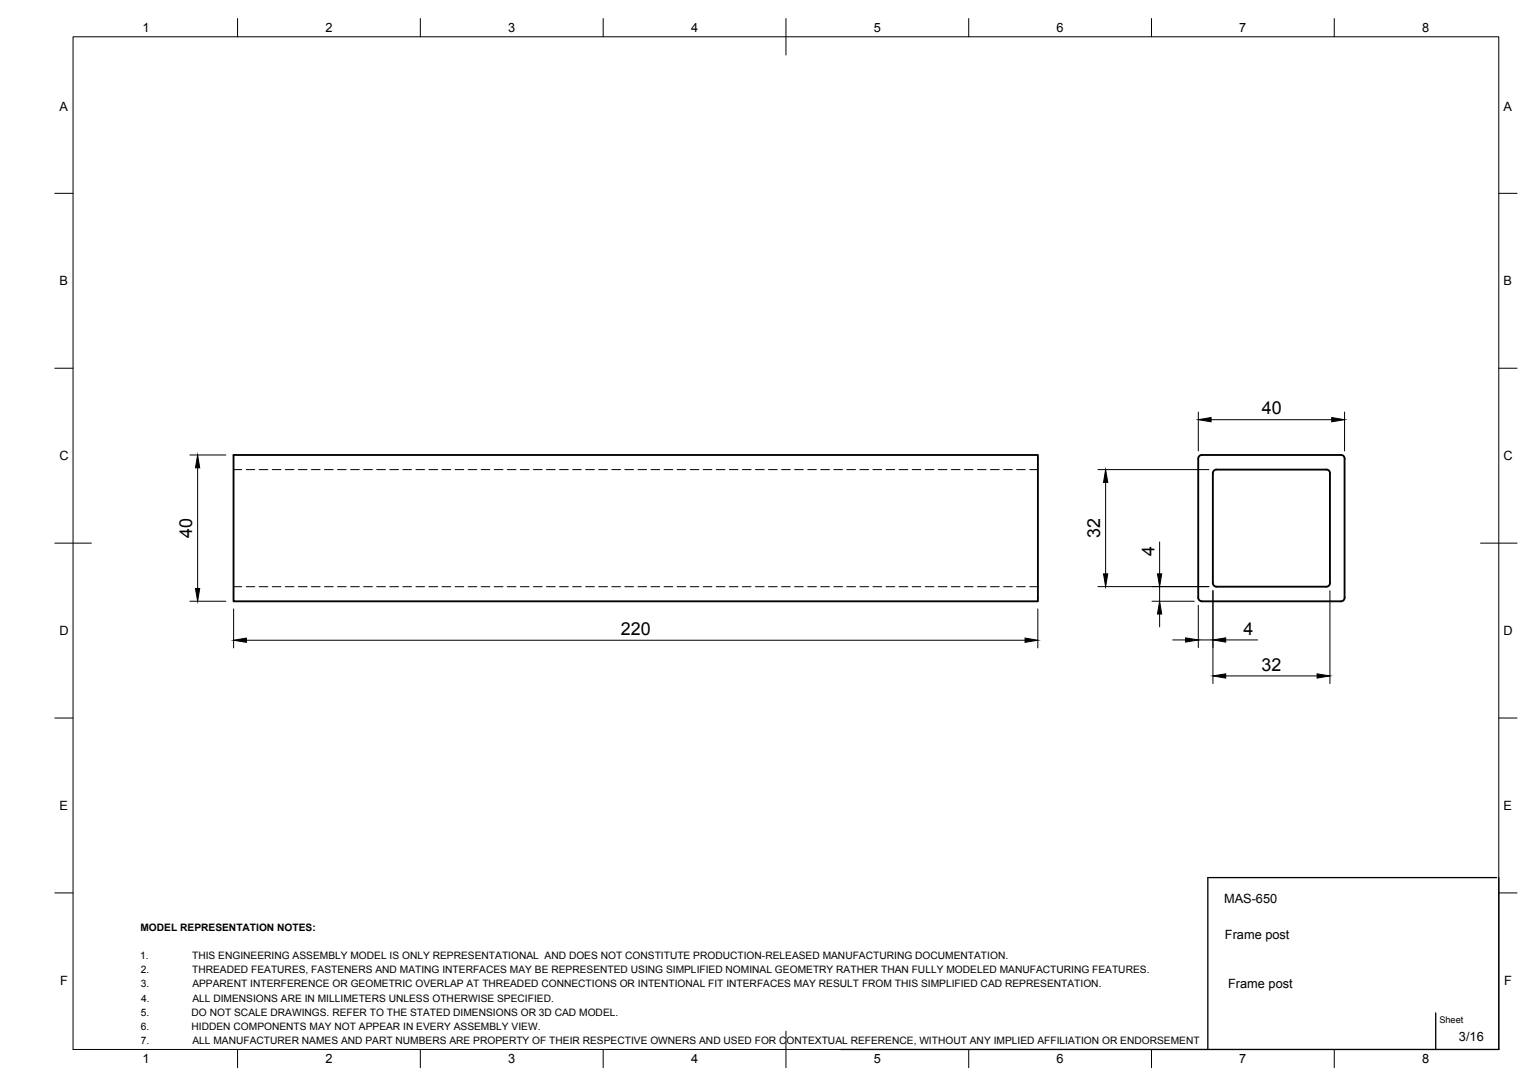
ISO-10303-21;
HEADER;
/* Generated by software containing ST-Developer
 * from STEP Tools, Inc. (www.steptools.com) 
 */

FILE_DESCRIPTION(
/* description */ ('Independent manual traversing gantry with native reusable aluminum pr
ofiles,180mm captured carriage travel, four bronze-bushed rollers, lin
ked ideal rolling motion, bonded acetal lateral guides, positive welde
d end stops and fully retained axle stacks. Editable native profile cu
t lengths220/400mm. Tool attachments viaM6 bridge-plate taps; mounted 
tool outside assembly. Welds, anchors, adhesives, fits, traction, load
/speed/structural/life ratings unassigned.'),
/* implementation_level */ '2;1');

FILE_NAME(
/* name */ 'Frame post.step',
/* time_stamp */ '2026-11-09T20:04:38-08:00',
/* author */ (''),
/* organization */ (''),
/* preprocessor_version */ 'ST-DEVELOPER v20.2',
/* originating_system */ 'Autodesk Translation Framework v15.17.0.0',
/* authorisation */ '');

FILE_SCHEMA (('AUTOMOTIVE_DESIGN { 1 0 10303 214 3 1 1 }'));
ENDSEC;

DATA;
#10=MECHANICAL_DESIGN_GEOMETRIC_PRESENTATION_REPRESENTATION('',(#472),#13231);
#440=SHAPE_REPRESENTATION_RELATIONSHIP('SRR','None',#13329,#456);
#456=ADVANCED_BREP_SHAPE_REPRESENTATION('',(#488),#13216);
#472=STYLED_ITEM('',(#13418),#488);
#488=MANIFOLD_SOLID_BREP('Aluminum square hollow profile',#4152);
#505=FACE_BOUND('',#877,.T.);
#506=FACE_BOUND('',#893,.T.);
#562=PLANE('',#4384);
#563=PLANE('',#4385);
#564=PLANE('',#4395);
#565=PLANE('',#4402);
#566=PLANE('',#4405);
#567=PLANE('',#4408);
#568=PLANE('',#4411);
#569=PLANE('',#4412);
#570=PLANE('',#4413);
#571=PLANE('',#4414);
#651=FACE_OUTER_BOUND('',#874,.T.);
#652=FACE_OUTER_BOUND('',#875,.T.);
#653=FACE_OUTER_BOUND('',#876,.T.);
#654=FACE_OUTER_BOUND('',#878,.T.);
#655=FACE_OUTER_BOUND('',#879,.T.);
#656=FACE_OUTER_BOUND('',#880,.T.);
#657=FACE_OUTER_BOUND('',#881,.T.);
#658=FACE_OUTER_BOUND('',#882,.T.);
#659=FACE_OUTER_BOUND('',#883,.T.);
#660=FACE_OUTER_BOUND('',#884,.T.);
#661=FACE_OUTER_BOUND('',#885,.T.);
#662=FACE_OUTER_BOUND('',#886,.T.);
#663=FACE_OUTER_BOUND('',#887,.T.);
#664=FACE_OUTER_BOUND('',#888,.T.);
#665=FACE_OUTER_BOUND('',#889,.T.);
#666=FACE_OUTER_BOUND('',#890,.T.);
#667=FACE_OUTER_BOUND('',#891,.T.);
#668=FACE_OUTER_BOUND('',#892,.T.);
#874=EDGE_LOOP('',(#2778,#2779,#2780,#2781));
#875=EDGE_LOOP('',(#2782,#2783,#2784,#2785));
#876=EDGE_LOOP('',(#2786,#2787,#2788,#2789,#2790,#2791,#2792,#2793));
#877=EDGE_LOOP('',(#2794,#2795,#2796,#2797,#2798,#2799,#2800,#2801));
#878=EDGE_LOOP('',(#2802,#2803,#2804,#2805));
#879=EDGE_LOOP('',(#2806,#2807,#2808,#2809));
#880=EDGE_LOOP('',(#2810,#2811,#2812,#2813));
#881=EDGE_LOOP('',(#2814,#2815,#2816,#2817));
#882=EDGE_LOOP('',(#2818,#2819,#2820,#2821));
#883=EDGE_LOOP('',(#2822,#2823,#2824,#2825));
#884=EDGE_LOOP('',(#2826,#2827,#2828,#2829));
#885=EDGE_LOOP('',(#2830,#2831,#2832,#2833));
#886=EDGE_LOOP('',(#2834,#2835,#2836,#2837));
#887=EDGE_LOOP('',(#2838,#2839,#2840,#2841));
#888=EDGE_LOOP('',(#2842,#2843,#2844,#2845));
#889=EDGE_LOOP('',(#2846,#2847,#2848,#2849));
#890=EDGE_LOOP('',(#2850,#2851,#2852,#2853));
#891=EDGE_LOOP('',(#2854,#2855,#2856,#2857));
#892=EDGE_LOOP('',(#2858,#2859,#2860,#2861,#2862,#2863,#2864,#2865));
#893=EDGE_LOOP('',(#2866,#2867,#2868,#2869,#2870,#2871,#2872,#2873));
#1156=LINE('',#5885,#1418);
#1157=LINE('',#5888,#1419);
#1158=LINE('',#5891,#1420);
#1159=LINE('',#5893,#1421);
#1160=LINE('',#5894,#1422);
#1161=LINE('',#5897,#1423);
#1162=LINE('',#5901,#1424);
#1163=LINE('',#5905,#1425);
#1164=LINE('',#5909,#1426);
#1165=LINE('',#5913,#1427);
#1166=LINE('',#5917,#1428);
#1167=LINE('',#5921,#1429);
#1168=LINE('',#5925,#1430);
#1169=LINE('',#5928,#1431);
#1170=LINE('',#5931,#1432);
#1171=LINE('',#5932,#1433);
#1172=LINE('',#5936,#1434);
#1173=LINE('',#5939,#1435);
#1174=LINE('',#5945,#1436);
#1175=LINE('',#5946,#1437);
#1176=LINE('',#5949,#1438);
#1177=LINE('',#5950,#1439);
#1178=LINE('',#5954,#1440);
#1179=LINE('',#5957,#1441);
#1180=LINE('',#5958,#1442);
#1181=LINE('',#5962,#1443);
#1182=LINE('',#5965,#1444);
#1183=LINE('',#5966,#1445);
#1184=LINE('',#5970,#1446);
#1185=LINE('',#5972,#1447);
#1186=LINE('',#5974,#1448);
#1187=LINE('',#5976,#1449);
#1418=VECTOR('',#4845,10.);
#1419=VECTOR('',#4848,10.);
#1420=VECTOR('',#4851,10.);
#1421=VECTOR('',#4852,10.);
#1422=VECTOR('',#4853,10.);
#1423=VECTOR('',#4856,10.);
#1424=VECTOR('',#4859,10.);
#1425=VECTOR('',#4862,10.);
#1426=VECTOR('',#4865,10.);
#1427=VECTOR('',#4868,10.);
#1428=VECTOR('',#4871,10.);
#1429=VECTOR('',#4874,10.);
#1430=VECTOR('',#4879,10.);
#1431=VECTOR('',#4882,10.);
#1432=VECTOR('',#4885,10.);
#1433=VECTOR('',#4886,10.);
#1434=VECTOR('',#4891,10.);
#1435=VECTOR('',#4894,10.);
#1436=VECTOR('',#4901,10.);
#1437=VECTOR('',#4902,10.);
#1438=VECTOR('',#4905,10.);
#1439=VECTOR('',#4906,10.);
#1440=VECTOR('',#4911,10.);
#1441=VECTOR('',#4914,10.);
#1442=VECTOR('',#4915,10.);
#1443=VECTOR('',#4920,10.);
#1444=VECTOR('',#4923,10.);
#1445=VECTOR('',#4924,10.);
#1446=VECTOR('',#4929,10.);
#1447=VECTOR('',#4932,10.);
#1448=VECTOR('',#4935,10.);
#1449=VECTOR('',#4938,10.);
#1664=CIRCLE('',#4382,1.);
#1665=CIRCLE('',#4383,1.);
#1666=CIRCLE('',#4386,1.);
#1667=CIRCLE('',#4387,1.);
#1668=CIRCLE('',#4388,1.);
#1669=CIRCLE('',#4389,1.);
#1670=CIRCLE('',#4390,1.);
#1671=CIRCLE('',#4391,1.);
#1672=CIRCLE('',#4392,1.);
#1673=CIRCLE('',#4394,1.);
#1674=CIRCLE('',#4397,1.);
#1675=CIRCLE('',#4399,1.);
#1676=CIRCLE('',#4401,1.);
#1677=CIRCLE('',#4404,1.);
#1678=CIRCLE('',#4407,1.);
#1679=CIRCLE('',#4410,1.);
#1784=VERTEX_POINT('',#5881);
#1785=VERTEX_POINT('',#5882);
#1786=VERTEX_POINT('',#5884);
#1787=VERTEX_POINT('',#5886);
#1788=VERTEX_POINT('',#5890);
#1789=VERTEX_POINT('',#5892);
#1790=VERTEX_POINT('',#5896);
#1791=VERTEX_POINT('',#5898);
#1792=VERTEX_POINT('',#5900);
#1793=VERTEX_POINT('',#5902);
#1794=VERTEX_POINT('',#5904);
#1795=VERTEX_POINT('',#5907);
#1796=VERTEX_POINT('',#5908);
#1797=VERTEX_POINT('',#5910);
#1798=VERTEX_POINT('',#5912);
#1799=VERTEX_POINT('',#5914);
#1800=VERTEX_POINT('',#5916);
#1801=VERTEX_POINT('',#5918);
#1802=VERTEX_POINT('',#5920);
#1803=VERTEX_POINT('',#5924);
#1804=VERTEX_POINT('',#5926);
#1805=VERTEX_POINT('',#5930);
#1806=VERTEX_POINT('',#5934);
#1807=VERTEX_POINT('',#5938);
#1808=VERTEX_POINT('',#5942);
#1809=VERTEX_POINT('',#5943);
#1810=VERTEX_POINT('',#5948);
#1811=VERTEX_POINT('',#5952);
#1812=VERTEX_POINT('',#5956);
#1813=VERTEX_POINT('',#5960);
#1814=VERTEX_POINT('',#5964);
#1815=VERTEX_POINT('',#5968);
#2172=EDGE_CURVE('',#1784,#1785,#1664,.T.);
#2173=EDGE_CURVE('',#1785,#1786,#1156,.T.);
#2174=EDGE_CURVE('',#1786,#1787,#1665,.T.);
#2175=EDGE_CURVE('',#1787,#1784,#1157,.T.);
#2176=EDGE_CURVE('',#1788,#1785,#1158,.T.);
#2177=EDGE_CURVE('',#1789,#1788,#1159,.T.);
#2178=EDGE_CURVE('',#1789,#1786,#1160,.T.);
#2179=EDGE_CURVE('',#1784,#1790,#1161,.T.);
#2180=EDGE_CURVE('',#1791,#1790,#1666,.T.);
#2181=EDGE_CURVE('',#1791,#1792,#1162,.T.);
#2182=EDGE_CURVE('',#1793,#1792,#1667,.T.);
#2183=EDGE_CURVE('',#1793,#1794,#1163,.T.);
#2184=EDGE_CURVE('',#1788,#1794,#1668,.T.);
#2185=EDGE_CURVE('',#1795,#1796,#1164,.T.);
#2186=EDGE_CURVE('',#1797,#1796,#1669,.T.);
#2187=EDGE_CURVE('',#1797,#1798,#1165,.T.);
#2188=EDGE_CURVE('',#1799,#1798,#1670,.T.);
#2189=EDGE_CURVE('',#1799,#1800,#1166,.T.);
#2190=EDGE_CURVE('',#1801,#1800,#1671,.T.);
#2191=EDGE_CURVE('',#1801,#1802,#1167,.T.);
#2192=EDGE_CURVE('',#1795,#1802,#1672,.T.);
#2193=EDGE_CURVE('',#1790,#1803,#1168,.T.);
#2194=EDGE_CURVE('',#1803,#1804,#1673,.T.);
#2195=EDGE_CURVE('',#1804,#1791,#1169,.T.);
#2196=EDGE_CURVE('',#1804,#1805,#1170,.T.);
#2197=EDGE_CURVE('',#1792,#1805,#1171,.T.);
#2198=EDGE_CURVE('',#1805,#1806,#1674,.T.);
#2199=EDGE_CURVE('',#1806,#1793,#1172,.T.);
#2200=EDGE_CURVE('',#1794,#1807,#1173,.T.);
#2201=EDGE_CURVE('',#1807,#1789,#1675,.T.);
#2202=EDGE_CURVE('',#1808,#1809,#1676,.T.);
#2203=EDGE_CURVE('',#1809,#1797,#1174,.T.);
#2204=EDGE_CURVE('',#1796,#1808,#1175,.T.);
#2205=EDGE_CURVE('',#1809,#1810,#1176,.T.);
#2206=EDGE_CURVE('',#1798,#1810,#1177,.T.);
#2207=EDGE_CURVE('',#1810,#1811,#1677,.T.);
#2208=EDGE_CURVE('',#1811,#1799,#1178,.T.);
#2209=EDGE_CURVE('',#1811,#1812,#1179,.T.);
#2210=EDGE_CURVE('',#1800,#1812,#1180,.T.);
#2211=EDGE_CURVE('',#1812,#1813,#1678,.T.);
#2212=EDGE_CURVE('',#1813,#1801,#1181,.T.);
#2213=EDGE_CURVE('',#1813,#1814,#1182,.T.);
#2214=EDGE_CURVE('',#1802,#1814,#1183,.T.);
#2215=EDGE_CURVE('',#1814,#1815,#1679,.T.);
#2216=EDGE_CURVE('',#1815,#1795,#1184,.T.);
#2217=EDGE_CURVE('',#1815,#1808,#1185,.T.);
#2218=EDGE_CURVE('',#1806,#1807,#1186,.T.);
#2219=EDGE_CURVE('',#1787,#1803,#1187,.T.);
#2778=ORIENTED_EDGE('',*,*,#2172,.T.);
#2779=ORIENTED_EDGE('',*,*,#2173,.T.);
#2780=ORIENTED_EDGE('',*,*,#2174,.T.);
#2781=ORIENTED_EDGE('',*,*,#2175,.T.);
#2782=ORIENTED_EDGE('',*,*,#2173,.F.);
#2783=ORIENTED_EDGE('',*,*,#2176,.F.);
#2784=ORIENTED_EDGE('',*,*,#2177,.F.);
#2785=ORIENTED_EDGE('',*,*,#2178,.T.);
#2786=ORIENTED_EDGE('',*,*,#2172,.F.);
#2787=ORIENTED_EDGE('',*,*,#2179,.T.);
#2788=ORIENTED_EDGE('',*,*,#2180,.F.);
#2789=ORIENTED_EDGE('',*,*,#2181,.T.);
#2790=ORIENTED_EDGE('',*,*,#2182,.F.);
#2791=ORIENTED_EDGE('',*,*,#2183,.T.);
#2792=ORIENTED_EDGE('',*,*,#2184,.F.);
#2793=ORIENTED_EDGE('',*,*,#2176,.T.);
#2794=ORIENTED_EDGE('',*,*,#2185,.T.);
#2795=ORIENTED_EDGE('',*,*,#2186,.F.);
#2796=ORIENTED_EDGE('',*,*,#2187,.T.);
#2797=ORIENTED_EDGE('',*,*,#2188,.F.);
#2798=ORIENTED_EDGE('',*,*,#2189,.T.);
#2799=ORIENTED_EDGE('',*,*,#2190,.F.);
#2800=ORIENTED_EDGE('',*,*,#2191,.T.);
#2801=ORIENTED_EDGE('',*,*,#2192,.F.);
#2802=ORIENTED_EDGE('',*,*,#2180,.T.);
#2803=ORIENTED_EDGE('',*,*,#2193,.T.);
#2804=ORIENTED_EDGE('',*,*,#2194,.T.);
#2805=ORIENTED_EDGE('',*,*,#2195,.T.);
#2806=ORIENTED_EDGE('',*,*,#2195,.F.);
#2807=ORIENTED_EDGE('',*,*,#2196,.T.);
#2808=ORIENTED_EDGE('',*,*,#2197,.F.);
#2809=ORIENTED_EDGE('',*,*,#2181,.F.);
#2810=ORIENTED_EDGE('',*,*,#2182,.T.);
#2811=ORIENTED_EDGE('',*,*,#2197,.T.);
#2812=ORIENTED_EDGE('',*,*,#2198,.T.);
#2813=ORIENTED_EDGE('',*,*,#2199,.T.);
#2814=ORIENTED_EDGE('',*,*,#2184,.T.);
#2815=ORIENTED_EDGE('',*,*,#2200,.T.);
#2816=ORIENTED_EDGE('',*,*,#2201,.T.);
#2817=ORIENTED_EDGE('',*,*,#2177,.T.);
#2818=ORIENTED_EDGE('',*,*,#2202,.T.);
#2819=ORIENTED_EDGE('',*,*,#2203,.T.);
#2820=ORIENTED_EDGE('',*,*,#2186,.T.);
#2821=ORIENTED_EDGE('',*,*,#2204,.T.);
#2822=ORIENTED_EDGE('',*,*,#2203,.F.);
#2823=ORIENTED_EDGE('',*,*,#2205,.T.);
#2824=ORIENTED_EDGE('',*,*,#2206,.F.);
#2825=ORIENTED_EDGE('',*,*,#2187,.F.);
#2826=ORIENTED_EDGE('',*,*,#2207,.T.);
#2827=ORIENTED_EDGE('',*,*,#2208,.T.);
#2828=ORIENTED_EDGE('',*,*,#2188,.T.);
#2829=ORIENTED_EDGE('',*,*,#2206,.T.);
#2830=ORIENTED_EDGE('',*,*,#2208,.F.);
#2831=ORIENTED_EDGE('',*,*,#2209,.T.);
#2832=ORIENTED_EDGE('',*,*,#2210,.F.);
#2833=ORIENTED_EDGE('',*,*,#2189,.F.);
#2834=ORIENTED_EDGE('',*,*,#2211,.T.);
#2835=ORIENTED_EDGE('',*,*,#2212,.T.);
#2836=ORIENTED_EDGE('',*,*,#2190,.T.);
#2837=ORIENTED_EDGE('',*,*,#2210,.T.);
#2838=ORIENTED_EDGE('',*,*,#2212,.F.);
#2839=ORIENTED_EDGE('',*,*,#2213,.T.);
#2840=ORIENTED_EDGE('',*,*,#2214,.F.);
#2841=ORIENTED_EDGE('',*,*,#2191,.F.);
#2842=ORIENTED_EDGE('',*,*,#2215,.T.);
#2843=ORIENTED_EDGE('',*,*,#2216,.T.);
#2844=ORIENTED_EDGE('',*,*,#2192,.T.);
#2845=ORIENTED_EDGE('',*,*,#2214,.T.);
#2846=ORIENTED_EDGE('',*,*,#2204,.F.);
#2847=ORIENTED_EDGE('',*,*,#2185,.F.);
#2848=ORIENTED_EDGE('',*,*,#2216,.F.);
#2849=ORIENTED_EDGE('',*,*,#2217,.T.);
#2850=ORIENTED_EDGE('',*,*,#2199,.F.);
#2851=ORIENTED_EDGE('',*,*,#2218,.T.);
#2852=ORIENTED_EDGE('',*,*,#2200,.F.);
#2853=ORIENTED_EDGE('',*,*,#2183,.F.);
#2854=ORIENTED_EDGE('',*,*,#2175,.F.);
#2855=ORIENTED_EDGE('',*,*,#2219,.T.);
#2856=ORIENTED_EDGE('',*,*,#2193,.F.);
#2857=ORIENTED_EDGE('',*,*,#2179,.F.);
#2858=ORIENTED_EDGE('',*,*,#2174,.F.);
#2859=ORIENTED_EDGE('',*,*,#2178,.F.);
#2860=ORIENTED_EDGE('',*,*,#2201,.F.);
#2861=ORIENTED_EDGE('',*,*,#2218,.F.);
#2862=ORIENTED_EDGE('',*,*,#2198,.F.);
#2863=ORIENTED_EDGE('',*,*,#2196,.F.);
#2864=ORIENTED_EDGE('',*,*,#2194,.F.);
#2865=ORIENTED_EDGE('',*,*,#2219,.F.);
#2866=ORIENTED_EDGE('',*,*,#2215,.F.);
#2867=ORIENTED_EDGE('',*,*,#2213,.F.);
#2868=ORIENTED_EDGE('',*,*,#2211,.F.);
#2869=ORIENTED_EDGE('',*,*,#2209,.F.);
#2870=ORIENTED_EDGE('',*,*,#2207,.F.);
#2871=ORIENTED_EDGE('',*,*,#2205,.F.);
#2872=ORIENTED_EDGE('',*,*,#2202,.F.);
#2873=ORIENTED_EDGE('',*,*,#2217,.F.);
#3806=CYLINDRICAL_SURFACE('',#4381,1.);
#3807=CYLINDRICAL_SURFACE('',#4393,1.);
#3808=CYLINDRICAL_SURFACE('',#4396,1.);
#3809=CYLINDRICAL_SURFACE('',#4398,1.);
#3810=CYLINDRICAL_SURFACE('',#4400,1.);
#3811=CYLINDRICAL_SURFACE('',#4403,1.);
#3812=CYLINDRICAL_SURFACE('',#4406,1.);
#3813=CYLINDRICAL_SURFACE('',#4409,1.);
#3948=ADVANCED_FACE('',(#651),#3806,.T.);
#3949=ADVANCED_FACE('',(#652),#562,.T.);
#3950=ADVANCED_FACE('',(#653,#505),#563,.T.);
#3951=ADVANCED_FACE('',(#654),#3807,.T.);
#3952=ADVANCED_FACE('',(#655),#564,.T.);
#3953=ADVANCED_FACE('',(#656),#3808,.T.);
#3954=ADVANCED_FACE('',(#657),#3809,.T.);
#3955=ADVANCED_FACE('',(#658),#3810,.F.);
#3956=ADVANCED_FACE('',(#659),#565,.T.);
#3957=ADVANCED_FACE('',(#660),#3811,.F.);
#3958=ADVANCED_FACE('',(#661),#566,.T.);
#3959=ADVANCED_FACE('',(#662),#3812,.F.);
#3960=ADVANCED_FACE('',(#663),#567,.T.);
#3961=ADVANCED_FACE('',(#664),#3813,.F.);
#3962=ADVANCED_FACE('',(#665),#568,.T.);
#3963=ADVANCED_FACE('',(#666),#569,.T.);
#3964=ADVANCED_FACE('',(#667),#570,.T.);
#3965=ADVANCED_FACE('',(#668,#506),#571,.F.);
#4152=CLOSED_SHELL('',(#3948,#3949,#3950,#3951,#3952,#3953,#3954,#3955,
#3956,#3957,#3958,#3959,#3960,#3961,#3962,#3963,#3964,#3965));
#4380=AXIS2_PLACEMENT_3D('',#5879,#4839,#4840);
#4381=AXIS2_PLACEMENT_3D('',#5880,#4841,#4842);
#4382=AXIS2_PLACEMENT_3D('',#5883,#4843,#4844);
#4383=AXIS2_PLACEMENT_3D('',#5887,#4846,#4847);
#4384=AXIS2_PLACEMENT_3D('',#5889,#4849,#4850);
#4385=AXIS2_PLACEMENT_3D('',#5895,#4854,#4855);
#4386=AXIS2_PLACEMENT_3D('',#5899,#4857,#4858);
#4387=AXIS2_PLACEMENT_3D('',#5903,#4860,#4861);
#4388=AXIS2_PLACEMENT_3D('',#5906,#4863,#4864);
#4389=AXIS2_PLACEMENT_3D('',#5911,#4866,#4867);
#4390=AXIS2_PLACEMENT_3D('',#5915,#4869,#4870);
#4391=AXIS2_PLACEMENT_3D('',#5919,#4872,#4873);
#4392=AXIS2_PLACEMENT_3D('',#5922,#4875,#4876);
#4393=AXIS2_PLACEMENT_3D('',#5923,#4877,#4878);
#4394=AXIS2_PLACEMENT_3D('',#5927,#4880,#4881);
#4395=AXIS2_PLACEMENT_3D('',#5929,#4883,#4884);
#4396=AXIS2_PLACEMENT_3D('',#5933,#4887,#4888);
#4397=AXIS2_PLACEMENT_3D('',#5935,#4889,#4890);
#4398=AXIS2_PLACEMENT_3D('',#5937,#4892,#4893);
#4399=AXIS2_PLACEMENT_3D('',#5940,#4895,#4896);
#4400=AXIS2_PLACEMENT_3D('',#5941,#4897,#4898);
#4401=AXIS2_PLACEMENT_3D('',#5944,#4899,#4900);
#4402=AXIS2_PLACEMENT_3D('',#5947,#4903,#4904);
#4403=AXIS2_PLACEMENT_3D('',#5951,#4907,#4908);
#4404=AXIS2_PLACEMENT_3D('',#5953,#4909,#4910);
#4405=AXIS2_PLACEMENT_3D('',#5955,#4912,#4913);
#4406=AXIS2_PLACEMENT_3D('',#5959,#4916,#4917);
#4407=AXIS2_PLACEMENT_3D('',#5961,#4918,#4919);
#4408=AXIS2_PLACEMENT_3D('',#5963,#4921,#4922);
#4409=AXIS2_PLACEMENT_3D('',#5967,#4925,#4926);
#4410=AXIS2_PLACEMENT_3D('',#5969,#4927,#4928);
#4411=AXIS2_PLACEMENT_3D('',#5971,#4930,#4931);
#4412=AXIS2_PLACEMENT_3D('',#5973,#4933,#4934);
#4413=AXIS2_PLACEMENT_3D('',#5975,#4936,#4937);
#4414=AXIS2_PLACEMENT_3D('',#5977,#4939,#4940);
#4839=DIRECTION('axis',(0.,0.,1.));
#4840=DIRECTION('refdir',(1.,0.,0.));
#4841=DIRECTION('center_axis',(0.,0.,1.));
#4842=DIRECTION('ref_axis',(-0.707106781186548,-0.707106781186548,0.));
#4843=DIRECTION('center_axis',(0.,0.,-1.));
#4844=DIRECTION('ref_axis',(-0.707106781186548,-0.707106781186548,0.));
#4845=DIRECTION('',(0.,0.,-1.));
#4846=DIRECTION('center_axis',(0.,0.,1.));
#4847=DIRECTION('ref_axis',(-0.707106781186548,-0.707106781186548,0.));
#4848=DIRECTION('',(0.,0.,1.));
#4849=DIRECTION('center_axis',(-1.,0.,0.));
#4850=DIRECTION('ref_axis',(0.,-1.,0.));
#4851=DIRECTION('',(0.,-1.,0.));
#4852=DIRECTION('',(0.,0.,1.));
#4853=DIRECTION('',(0.,-1.,0.));
#4854=DIRECTION('center_axis',(0.,0.,1.));
#4855=DIRECTION('ref_axis',(1.,0.,0.));
#4856=DIRECTION('',(1.,0.,0.));
#4857=DIRECTION('center_axis',(0.,0.,-1.));
#4858=DIRECTION('ref_axis',(0.707106781186548,-0.707106781186548,0.));
#4859=DIRECTION('',(0.,1.,0.));
#4860=DIRECTION('center_axis',(0.,0.,-1.));
#4861=DIRECTION('ref_axis',(0.707106781186548,0.707106781186548,0.));
#4862=DIRECTION('',(-1.,0.,0.));
#4863=DIRECTION('center_axis',(0.,0.,-1.));
#4864=DIRECTION('ref_axis',(-0.707106781186548,0.707106781186548,0.));
#4865=DIRECTION('',(0.,1.,0.));
#4866=DIRECTION('center_axis',(0.,0.,1.));
#4867=DIRECTION('ref_axis',(-0.707106781186548,0.707106781186548,0.));
#4868=DIRECTION('',(1.,0.,0.));
#4869=DIRECTION('center_axis',(0.,0.,1.));
#4870=DIRECTION('ref_axis',(0.707106781186548,0.707106781186548,0.));
#4871=DIRECTION('',(0.,-1.,0.));
#4872=DIRECTION('center_axis',(0.,0.,1.));
#4873=DIRECTION('ref_axis',(0.707106781186548,-0.707106781186548,0.));
#4874=DIRECTION('',(-1.,0.,0.));
#4875=DIRECTION('center_axis',(0.,0.,1.));
#4876=DIRECTION('ref_axis',(-0.707106781186548,-0.707106781186548,0.));
#4877=DIRECTION('center_axis',(0.,0.,1.));
#4878=DIRECTION('ref_axis',(0.707106781186548,-0.707106781186548,0.));
#4879=DIRECTION('',(0.,0.,-1.));
#4880=DIRECTION('center_axis',(0.,0.,1.));
#4881=DIRECTION('ref_axis',(0.707106781186548,-0.707106781186548,0.));
#4882=DIRECTION('',(0.,0.,1.));
#4883=DIRECTION('center_axis',(1.,0.,0.));
#4884=DIRECTION('ref_axis',(0.,1.,0.));
#4885=DIRECTION('',(0.,1.,0.));
#4886=DIRECTION('',(0.,0.,-1.));
#4887=DIRECTION('center_axis',(0.,0.,1.));
#4888=DIRECTION('ref_axis',(0.707106781186548,0.707106781186548,0.));
#4889=DIRECTION('center_axis',(0.,0.,1.));
#4890=DIRECTION('ref_axis',(0.707106781186548,0.707106781186548,0.));
#4891=DIRECTION('',(0.,0.,1.));
#4892=DIRECTION('center_axis',(0.,0.,1.));
#4893=DIRECTION('ref_axis',(-0.707106781186548,0.707106781186548,0.));
#4894=DIRECTION('',(0.,0.,-1.));
#4895=DIRECTION('center_axis',(0.,0.,1.));
#4896=DIRECTION('ref_axis',(-0.707106781186548,0.707106781186548,0.));
#4897=DIRECTION('center_axis',(0.,0.,1.));
#4898=DIRECTION('ref_axis',(-0.707106781186548,0.707106781186548,0.));
#4899=DIRECTION('center_axis',(0.,0.,-1.));
#4900=DIRECTION('ref_axis',(-0.707106781186548,0.707106781186548,0.));
#4901=DIRECTION('',(0.,0.,1.));
#4902=DIRECTION('',(0.,0.,-1.));
#4903=DIRECTION('center_axis',(0.,-1.,0.));
#4904=DIRECTION('ref_axis',(1.,0.,0.));
#4905=DIRECTION('',(1.,0.,0.));
#4906=DIRECTION('',(0.,0.,-1.));
#4907=DIRECTION('center_axis',(0.,0.,1.));
#4908=DIRECTION('ref_axis',(0.707106781186548,0.707106781186548,0.));
#4909=DIRECTION('center_axis',(0.,0.,-1.));
#4910=DIRECTION('ref_axis',(0.707106781186548,0.707106781186548,0.));
#4911=DIRECTION('',(0.,0.,1.));
#4912=DIRECTION('center_axis',(-1.,0.,0.));
#4913=DIRECTION('ref_axis',(0.,-1.,0.));
#4914=DIRECTION('',(0.,-1.,0.));
#4915=DIRECTION('',(0.,0.,-1.));
#4916=DIRECTION('center_axis',(0.,0.,1.));
#4917=DIRECTION('ref_axis',(0.707106781186548,-0.707106781186548,0.));
#4918=DIRECTION('center_axis',(0.,0.,-1.));
#4919=DIRECTION('ref_axis',(0.707106781186548,-0.707106781186548,0.));
#4920=DIRECTION('',(0.,0.,1.));
#4921=DIRECTION('center_axis',(0.,1.,0.));
#4922=DIRECTION('ref_axis',(-1.,0.,0.));
#4923=DIRECTION('',(-1.,0.,0.));
#4924=DIRECTION('',(0.,0.,-1.));
#4925=DIRECTION('center_axis',(0.,0.,1.));
#4926=DIRECTION('ref_axis',(-0.707106781186548,-0.707106781186548,0.));
#4927=DIRECTION('center_axis',(0.,0.,-1.));
#4928=DIRECTION('ref_axis',(-0.707106781186548,-0.707106781186548,0.));
#4929=DIRECTION('',(0.,0.,1.));
#4930=DIRECTION('center_axis',(1.,0.,0.));
#4931=DIRECTION('ref_axis',(0.,1.,0.));
#4932=DIRECTION('',(0.,1.,0.));
#4933=DIRECTION('center_axis',(0.,1.,0.));
#4934=DIRECTION('ref_axis',(-1.,0.,0.));
#4935=DIRECTION('',(-1.,0.,0.));
#4936=DIRECTION('center_axis',(0.,-1.,0.));
#4937=DIRECTION('ref_axis',(1.,0.,0.));
#4938=DIRECTION('',(1.,0.,0.));
#4939=DIRECTION('center_axis',(0.,0.,1.));
#4940=DIRECTION('ref_axis',(1.,0.,0.));
#5879=CARTESIAN_POINT('',(0.,0.,0.));
#5880=CARTESIAN_POINT('Origin',(-19.,-19.,0.));
#5881=CARTESIAN_POINT('',(-19.,-20.,220.));
#5882=CARTESIAN_POINT('',(-20.,-19.,220.));
#5883=CARTESIAN_POINT('Origin',(-19.,-19.,220.));
#5884=CARTESIAN_POINT('',(-20.,-19.,0.));
#5885=CARTESIAN_POINT('',(-20.,-19.,0.));
#5886=CARTESIAN_POINT('',(-19.,-20.,0.));
#5887=CARTESIAN_POINT('Origin',(-19.,-19.,0.));
#5888=CARTESIAN_POINT('',(-19.,-20.,0.));
#5889=CARTESIAN_POINT('Origin',(-20.,20.,0.));
#5890=CARTESIAN_POINT('',(-20.,19.,220.));
#5891=CARTESIAN_POINT('',(-20.,20.,220.));
#5892=CARTESIAN_POINT('',(-20.,19.,0.));
#5893=CARTESIAN_POINT('',(-20.,19.,0.));
#5894=CARTESIAN_POINT('',(-20.,20.,0.));
#5895=CARTESIAN_POINT('Origin',(0.,0.,220.));
#5896=CARTESIAN_POINT('',(19.,-20.,220.));
#5897=CARTESIAN_POINT('',(-20.,-20.,220.));
#5898=CARTESIAN_POINT('',(20.,-19.,220.));
#5899=CARTESIAN_POINT('Origin',(19.,-19.,220.));
#5900=CARTESIAN_POINT('',(20.,19.,220.));
#5901=CARTESIAN_POINT('',(20.,-20.,220.));
#5902=CARTESIAN_POINT('',(19.,20.,220.));
#5903=CARTESIAN_POINT('Origin',(19.,19.,220.));
#5904=CARTESIAN_POINT('',(-19.,20.,220.));
#5905=CARTESIAN_POINT('',(20.,20.,220.));
#5906=CARTESIAN_POINT('Origin',(-19.,19.,220.));
#5907=CARTESIAN_POINT('',(-16.,-15.,220.));
#5908=CARTESIAN_POINT('',(-16.,15.,220.));
#5909=CARTESIAN_POINT('',(-16.,16.,220.));
#5910=CARTESIAN_POINT('',(-15.,16.,220.));
#5911=CARTESIAN_POINT('Origin',(-15.,15.,220.));
#5912=CARTESIAN_POINT('',(15.,16.,220.));
#5913=CARTESIAN_POINT('',(16.,16.,220.));
#5914=CARTESIAN_POINT('',(16.,15.,220.));
#5915=CARTESIAN_POINT('Origin',(15.,15.,220.));
#5916=CARTESIAN_POINT('',(16.,-15.,220.));
#5917=CARTESIAN_POINT('',(16.,-16.,220.));
#5918=CARTESIAN_POINT('',(15.,-16.,220.));
#5919=CARTESIAN_POINT('Origin',(15.,-15.,220.));
#5920=CARTESIAN_POINT('',(-15.,-16.,220.));
#5921=CARTESIAN_POINT('',(-16.,-16.,220.));
#5922=CARTESIAN_POINT('Origin',(-15.,-15.,220.));
#5923=CARTESIAN_POINT('Origin',(19.,-19.,0.));
#5924=CARTESIAN_POINT('',(19.,-20.,0.));
#5925=CARTESIAN_POINT('',(19.,-20.,0.));
#5926=CARTESIAN_POINT('',(20.,-19.,0.));
#5927=CARTESIAN_POINT('Origin',(19.,-19.,0.));
#5928=CARTESIAN_POINT('',(20.,-19.,0.));
#5929=CARTESIAN_POINT('Origin',(20.,-20.,0.));
#5930=CARTESIAN_POINT('',(20.,19.,0.));
#5931=CARTESIAN_POINT('',(20.,-20.,0.));
#5932=CARTESIAN_POINT('',(20.,19.,0.));
#5933=CARTESIAN_POINT('Origin',(19.,19.,0.));
#5934=CARTESIAN_POINT('',(19.,20.,0.));
#5935=CARTESIAN_POINT('Origin',(19.,19.,0.));
#5936=CARTESIAN_POINT('',(19.,20.,0.));
#5937=CARTESIAN_POINT('Origin',(-19.,19.,0.));
#5938=CARTESIAN_POINT('',(-19.,20.,0.));
#5939=CARTESIAN_POINT('',(-19.,20.,0.));
#5940=CARTESIAN_POINT('Origin',(-19.,19.,0.));
#5941=CARTESIAN_POINT('Origin',(-15.,15.,0.));
#5942=CARTESIAN_POINT('',(-16.,15.,0.));
#5943=CARTESIAN_POINT('',(-15.,16.,0.));
#5944=CARTESIAN_POINT('Origin',(-15.,15.,0.));
#5945=CARTESIAN_POINT('',(-15.,16.,0.));
#5946=CARTESIAN_POINT('',(-16.,15.,0.));
#5947=CARTESIAN_POINT('Origin',(-16.,16.,0.));
#5948=CARTESIAN_POINT('',(15.,16.,0.));
#5949=CARTESIAN_POINT('',(16.,16.,0.));
#5950=CARTESIAN_POINT('',(15.,16.,0.));
#5951=CARTESIAN_POINT('Origin',(15.,15.,0.));
#5952=CARTESIAN_POINT('',(16.,15.,0.));
#5953=CARTESIAN_POINT('Origin',(15.,15.,0.));
#5954=CARTESIAN_POINT('',(16.,15.,0.));
#5955=CARTESIAN_POINT('Origin',(16.,16.,0.));
#5956=CARTESIAN_POINT('',(16.,-15.,0.));
#5957=CARTESIAN_POINT('',(16.,-16.,0.));
#5958=CARTESIAN_POINT('',(16.,-15.,0.));
#5959=CARTESIAN_POINT('Origin',(15.,-15.,0.));
#5960=CARTESIAN_POINT('',(15.,-16.,0.));
#5961=CARTESIAN_POINT('Origin',(15.,-15.,0.));
#5962=CARTESIAN_POINT('',(15.,-16.,0.));
#5963=CARTESIAN_POINT('Origin',(16.,-16.,0.));
#5964=CARTESIAN_POINT('',(-15.,-16.,0.));
#5965=CARTESIAN_POINT('',(-16.,-16.,0.));
#5966=CARTESIAN_POINT('',(-15.,-16.,0.));
#5967=CARTESIAN_POINT('Origin',(-15.,-15.,0.));
#5968=CARTESIAN_POINT('',(-16.,-15.,0.));
#5969=CARTESIAN_POINT('Origin',(-15.,-15.,0.));
#5970=CARTESIAN_POINT('',(-16.,-15.,0.));
#5971=CARTESIAN_POINT('Origin',(-16.,-16.,0.));
#5972=CARTESIAN_POINT('',(-16.,16.,0.));
#5973=CARTESIAN_POINT('Origin',(20.,20.,0.));
#5974=CARTESIAN_POINT('',(20.,20.,0.));
#5975=CARTESIAN_POINT('Origin',(-20.,-20.,0.));
#5976=CARTESIAN_POINT('',(-20.,-20.,0.));
#5977=CARTESIAN_POINT('Origin',(0.,0.,0.));
#13198=UNCERTAINTY_MEASURE_WITH_UNIT(LENGTH_MEASURE(0.01),#13232,
'DISTANCE_ACCURACY_VALUE',
'Maximum model space distance between geometric entities at asserted c
onnectivities');
#13213=UNCERTAINTY_MEASURE_WITH_UNIT(LENGTH_MEASURE(0.01),#13232,
'DISTANCE_ACCURACY_VALUE',
'Maximum model space distance between geometric entities at asserted c
onnectivities');
#13216=(
GEOMETRIC_REPRESENTATION_CONTEXT(3)
GLOBAL_UNCERTAINTY_ASSIGNED_CONTEXT((#13198))
GLOBAL_UNIT_ASSIGNED_CONTEXT((#13232,#13234,#13235))
REPRESENTATION_CONTEXT('','3D')
);
#13231=(
GEOMETRIC_REPRESENTATION_CONTEXT(3)
GLOBAL_UNCERTAINTY_ASSIGNED_CONTEXT((#13213))
GLOBAL_UNIT_ASSIGNED_CONTEXT((#13232,#13234,#13235))
REPRESENTATION_CONTEXT('','3D')
);
#13232=(
LENGTH_UNIT()
NAMED_UNIT(*)
SI_UNIT(.MILLI.,.METRE.)
);
#13234=(
NAMED_UNIT(*)
PLANE_ANGLE_UNIT()
SI_UNIT($,.RADIAN.)
);
#13235=(
NAMED_UNIT(*)
SI_UNIT($,.STERADIAN.)
SOLID_ANGLE_UNIT()
);
#13238=SHAPE_DEFINITION_REPRESENTATION(#13255,#13329);
#13255=PRODUCT_DEFINITION_SHAPE('',$,#13347);
#13329=SHAPE_REPRESENTATION('',(#4380),#13216);
#13344=PRODUCT_DEFINITION_CONTEXT('part definition',#13397,'design');
#13347=PRODUCT_DEFINITION('Frame post','Frame post',#13364,#13344);
#13364=PRODUCT_DEFINITION_FORMATION('',$,#13401);
#13397=APPLICATION_CONTEXT(
'Core Data for Automotive Mechanical Design Process');
#13398=PRODUCT_CONTEXT('part definition',#13397,'mechanical');
#13401=PRODUCT('Frame post','Frame post',
'Independent aluminum extrusion section. Whole-mm nominal die dimensio
ns; parametric saw-cut length. Select structural loading, tolerances a
nd finish for the assembly application.',(#13398));
#13418=PRESENTATION_STYLE_ASSIGNMENT((#13432));
#13432=SURFACE_STYLE_USAGE(.BOTH.,#13446);
#13446=SURFACE_SIDE_STYLE('',(#13460));
#13460=SURFACE_STYLE_FILL_AREA(#13474);
#13474=FILL_AREA_STYLE('Post gray',(#13488));
#13488=FILL_AREA_STYLE_COLOUR('Post gray',#13502);
#13502=COLOUR_RGB('Post gray',0.407843137254902,0.447058823529412,0.498039215686275);
ENDSEC;
END-ISO-10303-21;
